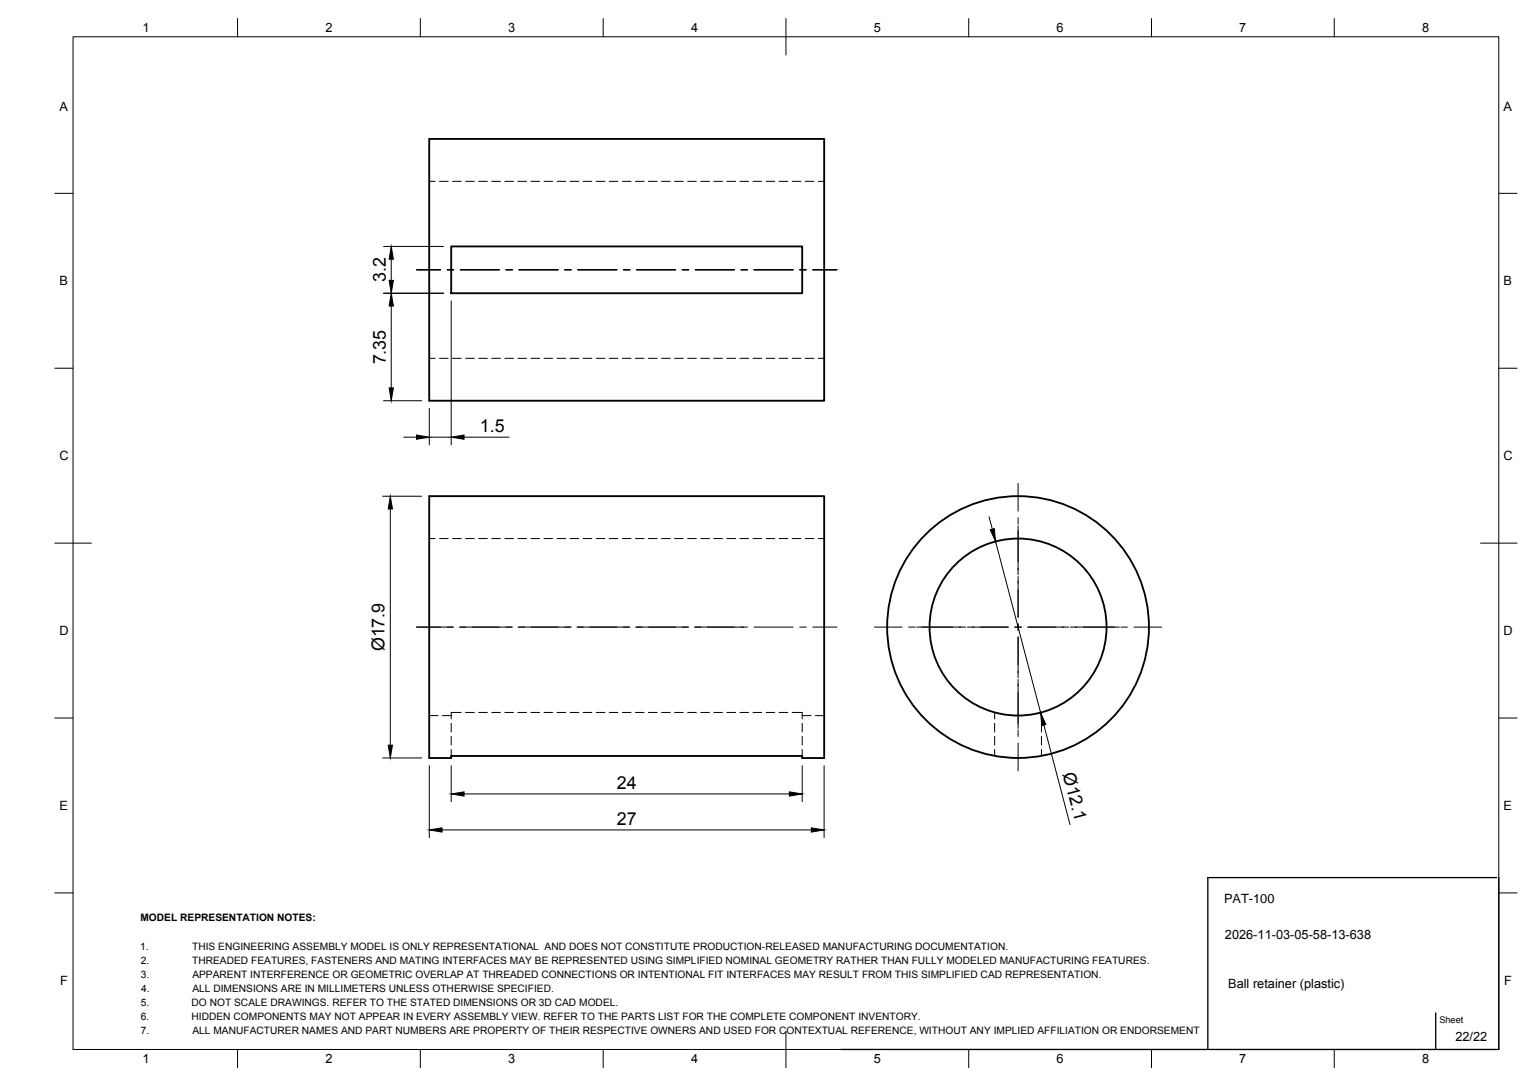
ISO-10303-21;
HEADER;
/* Generated by software containing ST-Developer
 * from STEP Tools, Inc. (www.steptools.com) 
 */

FILE_DESCRIPTION(
/* description */ (''),
/* implementation_level */ '2;1');

FILE_NAME(
/* name */ 'Ball retainer (plastic).step',
/* time_stamp */ '2026-10-29T16:43:51-07:00',
/* author */ (''),
/* organization */ (''),
/* preprocessor_version */ 'ST-DEVELOPER v20.2',
/* originating_system */ 'Autodesk Translation Framework v15.17.0.0',
/* authorisation */ '');

FILE_SCHEMA (('AUTOMOTIVE_DESIGN { 1 0 10303 214 3 1 1 }'));
ENDSEC;

DATA;
#10=MECHANICAL_DESIGN_GEOMETRIC_PRESENTATION_REPRESENTATION('',(#381),#10292);
#335=SHAPE_REPRESENTATION_RELATIONSHIP('SRR','None',#10433,#358);
#358=ADVANCED_BREP_SHAPE_REPRESENTATION('',(#402),#10285);
#381=STYLED_ITEM('',(#10621),#402);
#402=MANIFOLD_SOLID_BREP('Body1',#5025);
#508=FACE_BOUND('',#1314,.T.);
#509=FACE_BOUND('',#1316,.T.);
#510=FACE_BOUND('',#1318,.T.);
#511=FACE_BOUND('',#1320,.T.);
#661=PLANE('',#5665);
#662=PLANE('',#5668);
#663=PLANE('',#5669);
#664=PLANE('',#5672);
#665=PLANE('',#5673);
#666=PLANE('',#5678);
#919=FACE_OUTER_BOUND('',#1309,.T.);
#920=FACE_OUTER_BOUND('',#1310,.T.);
#921=FACE_OUTER_BOUND('',#1311,.T.);
#922=FACE_OUTER_BOUND('',#1312,.T.);
#923=FACE_OUTER_BOUND('',#1313,.T.);
#924=FACE_OUTER_BOUND('',#1315,.T.);
#925=FACE_OUTER_BOUND('',#1317,.T.);
#926=FACE_OUTER_BOUND('',#1319,.T.);
#1309=EDGE_LOOP('',(#4325,#4326,#4327,#4328));
#1310=EDGE_LOOP('',(#4329,#4330,#4331,#4332));
#1311=EDGE_LOOP('',(#4333,#4334,#4335,#4336));
#1312=EDGE_LOOP('',(#4337,#4338,#4339,#4340));
#1313=EDGE_LOOP('',(#4341));
#1314=EDGE_LOOP('',(#4342));
#1315=EDGE_LOOP('',(#4343,#4344,#4345,#4346));
#1316=EDGE_LOOP('',(#4347,#4348,#4349,#4350));
#1317=EDGE_LOOP('',(#4351));
#1318=EDGE_LOOP('',(#4352));
#1319=EDGE_LOOP('',(#4353,#4354,#4355,#4356));
#1320=EDGE_LOOP('',(#4357,#4358,#4359,#4360));
#1699=LINE('',#9839,#2091);
#1700=LINE('',#9842,#2092);
#1701=LINE('',#9845,#2093);
#1702=LINE('',#9847,#2094);
#1703=LINE('',#9848,#2095);
#1704=LINE('',#9854,#2096);
#1705=LINE('',#9856,#2097);
#1706=LINE('',#9857,#2098);
#1707=LINE('',#9866,#2099);
#1708=LINE('',#9871,#2100);
#2091=VECTOR('',#6908,1.);
#2092=VECTOR('',#6911,1.);
#2093=VECTOR('',#6914,1.);
#2094=VECTOR('',#6915,1.);
#2095=VECTOR('',#6916,1.);
#2096=VECTOR('',#6923,1.);
#2097=VECTOR('',#6926,1.);
#2098=VECTOR('',#6927,1.);
#2099=VECTOR('',#6938,0.895);
#2100=VECTOR('',#6945,0.605);
#2342=CIRCLE('',#5666,0.895);
#2343=CIRCLE('',#5667,0.605);
#2344=CIRCLE('',#5670,0.895);
#2345=CIRCLE('',#5671,0.605);
#2346=CIRCLE('',#5674,0.895);
#2347=CIRCLE('',#5675,0.605);
#2348=CIRCLE('',#5677,0.895);
#2349=CIRCLE('',#5679,0.605);
#2695=VERTEX_POINT('',#9835);
#2696=VERTEX_POINT('',#9836);
#2697=VERTEX_POINT('',#9838);
#2698=VERTEX_POINT('',#9840);
#2699=VERTEX_POINT('',#9844);
#2700=VERTEX_POINT('',#9846);
#2701=VERTEX_POINT('',#9850);
#2702=VERTEX_POINT('',#9852);
#2703=VERTEX_POINT('',#9859);
#2704=VERTEX_POINT('',#9861);
#2705=VERTEX_POINT('',#9864);
#2706=VERTEX_POINT('',#9868);
#3253=EDGE_CURVE('',#2695,#2696,#2342,.T.);
#3254=EDGE_CURVE('',#2697,#2695,#1699,.T.);
#3255=EDGE_CURVE('',#2698,#2697,#2343,.T.);
#3256=EDGE_CURVE('',#2696,#2698,#1700,.T.);
#3257=EDGE_CURVE('',#2696,#2699,#1701,.T.);
#3258=EDGE_CURVE('',#2700,#2698,#1702,.T.);
#3259=EDGE_CURVE('',#2700,#2699,#1703,.T.);
#3260=EDGE_CURVE('',#2699,#2701,#2344,.T.);
#3261=EDGE_CURVE('',#2702,#2700,#2345,.T.);
#3262=EDGE_CURVE('',#2701,#2702,#1704,.T.);
#3263=EDGE_CURVE('',#2701,#2695,#1705,.T.);
#3264=EDGE_CURVE('',#2697,#2702,#1706,.T.);
#3265=EDGE_CURVE('',#2703,#2703,#2346,.T.);
#3266=EDGE_CURVE('',#2704,#2704,#2347,.T.);
#3267=EDGE_CURVE('',#2705,#2705,#2348,.T.);
#3268=EDGE_CURVE('',#2705,#2703,#1707,.T.);
#3269=EDGE_CURVE('',#2706,#2706,#2349,.T.);
#3270=EDGE_CURVE('',#2706,#2704,#1708,.T.);
#4325=ORIENTED_EDGE('',*,*,#3253,.F.);
#4326=ORIENTED_EDGE('',*,*,#3254,.F.);
#4327=ORIENTED_EDGE('',*,*,#3255,.F.);
#4328=ORIENTED_EDGE('',*,*,#3256,.F.);
#4329=ORIENTED_EDGE('',*,*,#3257,.F.);
#4330=ORIENTED_EDGE('',*,*,#3256,.T.);
#4331=ORIENTED_EDGE('',*,*,#3258,.F.);
#4332=ORIENTED_EDGE('',*,*,#3259,.T.);
#4333=ORIENTED_EDGE('',*,*,#3260,.F.);
#4334=ORIENTED_EDGE('',*,*,#3259,.F.);
#4335=ORIENTED_EDGE('',*,*,#3261,.F.);
#4336=ORIENTED_EDGE('',*,*,#3262,.F.);
#4337=ORIENTED_EDGE('',*,*,#3263,.F.);
#4338=ORIENTED_EDGE('',*,*,#3262,.T.);
#4339=ORIENTED_EDGE('',*,*,#3264,.F.);
#4340=ORIENTED_EDGE('',*,*,#3254,.T.);
#4341=ORIENTED_EDGE('',*,*,#3265,.F.);
#4342=ORIENTED_EDGE('',*,*,#3266,.T.);
#4343=ORIENTED_EDGE('',*,*,#3267,.F.);
#4344=ORIENTED_EDGE('',*,*,#3268,.T.);
#4345=ORIENTED_EDGE('',*,*,#3265,.T.);
#4346=ORIENTED_EDGE('',*,*,#3268,.F.);
#4347=ORIENTED_EDGE('',*,*,#3260,.T.);
#4348=ORIENTED_EDGE('',*,*,#3263,.T.);
#4349=ORIENTED_EDGE('',*,*,#3253,.T.);
#4350=ORIENTED_EDGE('',*,*,#3257,.T.);
#4351=ORIENTED_EDGE('',*,*,#3267,.T.);
#4352=ORIENTED_EDGE('',*,*,#3269,.F.);
#4353=ORIENTED_EDGE('',*,*,#3269,.T.);
#4354=ORIENTED_EDGE('',*,*,#3270,.T.);
#4355=ORIENTED_EDGE('',*,*,#3266,.F.);
#4356=ORIENTED_EDGE('',*,*,#3270,.F.);
#4357=ORIENTED_EDGE('',*,*,#3261,.T.);
#4358=ORIENTED_EDGE('',*,*,#3258,.T.);
#4359=ORIENTED_EDGE('',*,*,#3255,.T.);
#4360=ORIENTED_EDGE('',*,*,#3264,.T.);
#4701=CYLINDRICAL_SURFACE('',#5676,0.895);
#4702=CYLINDRICAL_SURFACE('',#5680,0.605);
#4928=ADVANCED_FACE('',(#919),#661,.F.);
#4929=ADVANCED_FACE('',(#920),#662,.F.);
#4930=ADVANCED_FACE('',(#921),#663,.F.);
#4931=ADVANCED_FACE('',(#922),#664,.F.);
#4932=ADVANCED_FACE('',(#923,#508),#665,.T.);
#4933=ADVANCED_FACE('',(#924,#509),#4701,.T.);
#4934=ADVANCED_FACE('',(#925,#510),#666,.T.);
#4935=ADVANCED_FACE('',(#926,#511),#4702,.F.);
#5025=CLOSED_SHELL('',(#4928,#4929,#4930,#4931,#4932,#4933,#4934,#4935));
#5664=AXIS2_PLACEMENT_3D('',#9833,#6902,#6903);
#5665=AXIS2_PLACEMENT_3D('',#9834,#6904,#6905);
#5666=AXIS2_PLACEMENT_3D('',#9837,#6906,#6907);
#5667=AXIS2_PLACEMENT_3D('',#9841,#6909,#6910);
#5668=AXIS2_PLACEMENT_3D('',#9843,#6912,#6913);
#5669=AXIS2_PLACEMENT_3D('',#9849,#6917,#6918);
#5670=AXIS2_PLACEMENT_3D('',#9851,#6919,#6920);
#5671=AXIS2_PLACEMENT_3D('',#9853,#6921,#6922);
#5672=AXIS2_PLACEMENT_3D('',#9855,#6924,#6925);
#5673=AXIS2_PLACEMENT_3D('',#9858,#6928,#6929);
#5674=AXIS2_PLACEMENT_3D('',#9860,#6930,#6931);
#5675=AXIS2_PLACEMENT_3D('',#9862,#6932,#6933);
#5676=AXIS2_PLACEMENT_3D('',#9863,#6934,#6935);
#5677=AXIS2_PLACEMENT_3D('',#9865,#6936,#6937);
#5678=AXIS2_PLACEMENT_3D('',#9867,#6939,#6940);
#5679=AXIS2_PLACEMENT_3D('',#9869,#6941,#6942);
#5680=AXIS2_PLACEMENT_3D('',#9870,#6943,#6944);
#6902=DIRECTION('axis',(0.,0.,1.));
#6903=DIRECTION('refdir',(1.,0.,0.));
#6904=DIRECTION('center_axis',(0.,1.,0.));
#6905=DIRECTION('ref_axis',(0.,0.,1.));
#6906=DIRECTION('center_axis',(0.,1.,0.));
#6907=DIRECTION('ref_axis',(1.,0.,0.));
#6908=DIRECTION('',(1.,0.,0.));
#6909=DIRECTION('center_axis',(0.,-1.,0.));
#6910=DIRECTION('ref_axis',(1.,0.,0.));
#6911=DIRECTION('',(-1.,0.,0.));
#6912=DIRECTION('center_axis',(0.,0.,-1.));
#6913=DIRECTION('ref_axis',(-1.,0.,0.));
#6914=DIRECTION('',(0.,-1.,0.));
#6915=DIRECTION('',(0.,1.,0.));
#6916=DIRECTION('',(1.,0.,0.));
#6917=DIRECTION('center_axis',(0.,-1.,0.));
#6918=DIRECTION('ref_axis',(0.,0.,-1.));
#6919=DIRECTION('center_axis',(0.,-1.,0.));
#6920=DIRECTION('ref_axis',(1.,0.,0.));
#6921=DIRECTION('center_axis',(0.,1.,0.));
#6922=DIRECTION('ref_axis',(1.,0.,0.));
#6923=DIRECTION('',(-1.,0.,0.));
#6924=DIRECTION('center_axis',(0.,0.,1.));
#6925=DIRECTION('ref_axis',(1.,0.,0.));
#6926=DIRECTION('',(0.,1.,0.));
#6927=DIRECTION('',(0.,-1.,0.));
#6928=DIRECTION('center_axis',(0.,1.,0.));
#6929=DIRECTION('ref_axis',(0.,0.,1.));
#6930=DIRECTION('center_axis',(0.,-1.,0.));
#6931=DIRECTION('ref_axis',(1.,0.,0.));
#6932=DIRECTION('center_axis',(0.,-1.,0.));
#6933=DIRECTION('ref_axis',(1.,0.,0.));
#6934=DIRECTION('center_axis',(0.,-1.,0.));
#6935=DIRECTION('ref_axis',(1.,0.,0.));
#6936=DIRECTION('center_axis',(0.,-1.,0.));
#6937=DIRECTION('ref_axis',(1.,0.,0.));
#6938=DIRECTION('',(0.,1.,0.));
#6939=DIRECTION('center_axis',(0.,-1.,0.));
#6940=DIRECTION('ref_axis',(0.,0.,-1.));
#6941=DIRECTION('center_axis',(0.,-1.,0.));
#6942=DIRECTION('ref_axis',(1.,0.,0.));
#6943=DIRECTION('center_axis',(0.,-1.,0.));
#6944=DIRECTION('ref_axis',(1.,0.,0.));
#6945=DIRECTION('',(0.,1.,0.));
#9833=CARTESIAN_POINT('',(0.,0.,0.));
#9834=CARTESIAN_POINT('Origin',(0.75,1.2,0.));
#9835=CARTESIAN_POINT('',(0.880582193778639,1.2,0.16));
#9836=CARTESIAN_POINT('',(0.880582193778639,1.2,-0.16));
#9837=CARTESIAN_POINT('Origin',(0.,1.2,0.));
#9838=CARTESIAN_POINT('',(0.583459510163302,1.2,0.16));
#9839=CARTESIAN_POINT('',(0.57,1.2,0.16));
#9840=CARTESIAN_POINT('',(0.583459510163302,1.2,-0.16));
#9841=CARTESIAN_POINT('Origin',(0.,1.2,0.));
#9842=CARTESIAN_POINT('',(0.93,1.2,-0.16));
#9843=CARTESIAN_POINT('Origin',(0.93,0.,-0.16));
#9844=CARTESIAN_POINT('',(0.880582193778639,-1.2,-0.16));
#9845=CARTESIAN_POINT('',(0.880582193778639,0.,-0.16));
#9846=CARTESIAN_POINT('',(0.583459510163302,-1.2,-0.16));
#9847=CARTESIAN_POINT('',(0.583459510163302,0.,-0.16));
#9848=CARTESIAN_POINT('',(0.93,-1.2,-0.16));
#9849=CARTESIAN_POINT('Origin',(0.75,-1.2,0.));
#9850=CARTESIAN_POINT('',(0.880582193778639,-1.2,0.16));
#9851=CARTESIAN_POINT('Origin',(0.,-1.2,0.));
#9852=CARTESIAN_POINT('',(0.583459510163302,-1.2,0.16));
#9853=CARTESIAN_POINT('Origin',(0.,-1.2,0.));
#9854=CARTESIAN_POINT('',(0.57,-1.2,0.16));
#9855=CARTESIAN_POINT('Origin',(0.57,0.,0.16));
#9856=CARTESIAN_POINT('',(0.880582193778639,0.,0.16));
#9857=CARTESIAN_POINT('',(0.583459510163302,0.,0.16));
#9858=CARTESIAN_POINT('Origin',(0.895,1.35,0.));
#9859=CARTESIAN_POINT('',(-0.895,1.35,-1.09605888523688E-16));
#9860=CARTESIAN_POINT('Origin',(0.,1.35,0.));
#9861=CARTESIAN_POINT('',(-0.605,1.35,-7.40911313484149E-17));
#9862=CARTESIAN_POINT('Origin',(0.,1.35,0.));
#9863=CARTESIAN_POINT('Origin',(0.,0.,0.));
#9864=CARTESIAN_POINT('',(-0.895,-1.35,-1.09605888523688E-16));
#9865=CARTESIAN_POINT('Origin',(0.,-1.35,0.));
#9866=CARTESIAN_POINT('',(-0.895,0.,-1.09605888523688E-16));
#9867=CARTESIAN_POINT('Origin',(0.605,-1.35,0.));
#9868=CARTESIAN_POINT('',(-0.605,-1.35,-7.40911313484149E-17));
#9869=CARTESIAN_POINT('Origin',(0.,-1.35,0.));
#9870=CARTESIAN_POINT('Origin',(0.,0.,0.));
#9871=CARTESIAN_POINT('',(-0.605,0.,-7.40911313484149E-17));
#10257=UNCERTAINTY_MEASURE_WITH_UNIT(LENGTH_MEASURE(0.001),#10293,
'DISTANCE_ACCURACY_VALUE',
'Maximum model space distance between geometric entities at asserted c
onnectivities');
#10264=UNCERTAINTY_MEASURE_WITH_UNIT(LENGTH_MEASURE(0.001),#10293,
'DISTANCE_ACCURACY_VALUE',
'Maximum model space distance between geometric entities at asserted c
onnectivities');
#10285=(
GEOMETRIC_REPRESENTATION_CONTEXT(3)
GLOBAL_UNCERTAINTY_ASSIGNED_CONTEXT((#10257))
GLOBAL_UNIT_ASSIGNED_CONTEXT((#10293,#10295,#10296))
REPRESENTATION_CONTEXT('','3D')
);
#10292=(
GEOMETRIC_REPRESENTATION_CONTEXT(3)
GLOBAL_UNCERTAINTY_ASSIGNED_CONTEXT((#10264))
GLOBAL_UNIT_ASSIGNED_CONTEXT((#10293,#10295,#10296))
REPRESENTATION_CONTEXT('','3D')
);
#10293=(
LENGTH_UNIT()
NAMED_UNIT(*)
SI_UNIT(.CENTI.,.METRE.)
);
#10295=(
NAMED_UNIT(*)
PLANE_ANGLE_UNIT()
SI_UNIT($,.RADIAN.)
);
#10296=(
NAMED_UNIT(*)
SI_UNIT($,.STERADIAN.)
SOLID_ANGLE_UNIT()
);
#10317=SHAPE_DEFINITION_REPRESENTATION(#10344,#10433);
#10344=PRODUCT_DEFINITION_SHAPE('',$,#10461);
#10433=SHAPE_REPRESENTATION('',(#5664),#10285);
#10440=PRODUCT_DEFINITION_CONTEXT('part definition',#10523,'design');
#10461=PRODUCT_DEFINITION('Ball retainer (plastic)',
'Ball retainer (plastic)',#10488,#10440);
#10488=PRODUCT_DEFINITION_FORMATION('',$,#10545);
#10523=APPLICATION_CONTEXT(
'Core Data for Automotive Mechanical Design Process');
#10524=PRODUCT_CONTEXT('part definition',#10523,'mechanical');
#10545=PRODUCT('Ball retainer (plastic)','Ball retainer (plastic)',
'Ball retainer (plastic)',(#10524));
#10615=COLOUR_RGB('Sky Blue',0.24,0.69,0.87);
#10616=FILL_AREA_STYLE_COLOUR('',#10615);
#10617=FILL_AREA_STYLE('',(#10616));
#10618=SURFACE_STYLE_FILL_AREA(#10617);
#10619=SURFACE_SIDE_STYLE('',(#10618));
#10620=SURFACE_STYLE_USAGE(.BOTH.,#10619);
#10621=PRESENTATION_STYLE_ASSIGNMENT((#10620));
ENDSEC;
END-ISO-10303-21;
